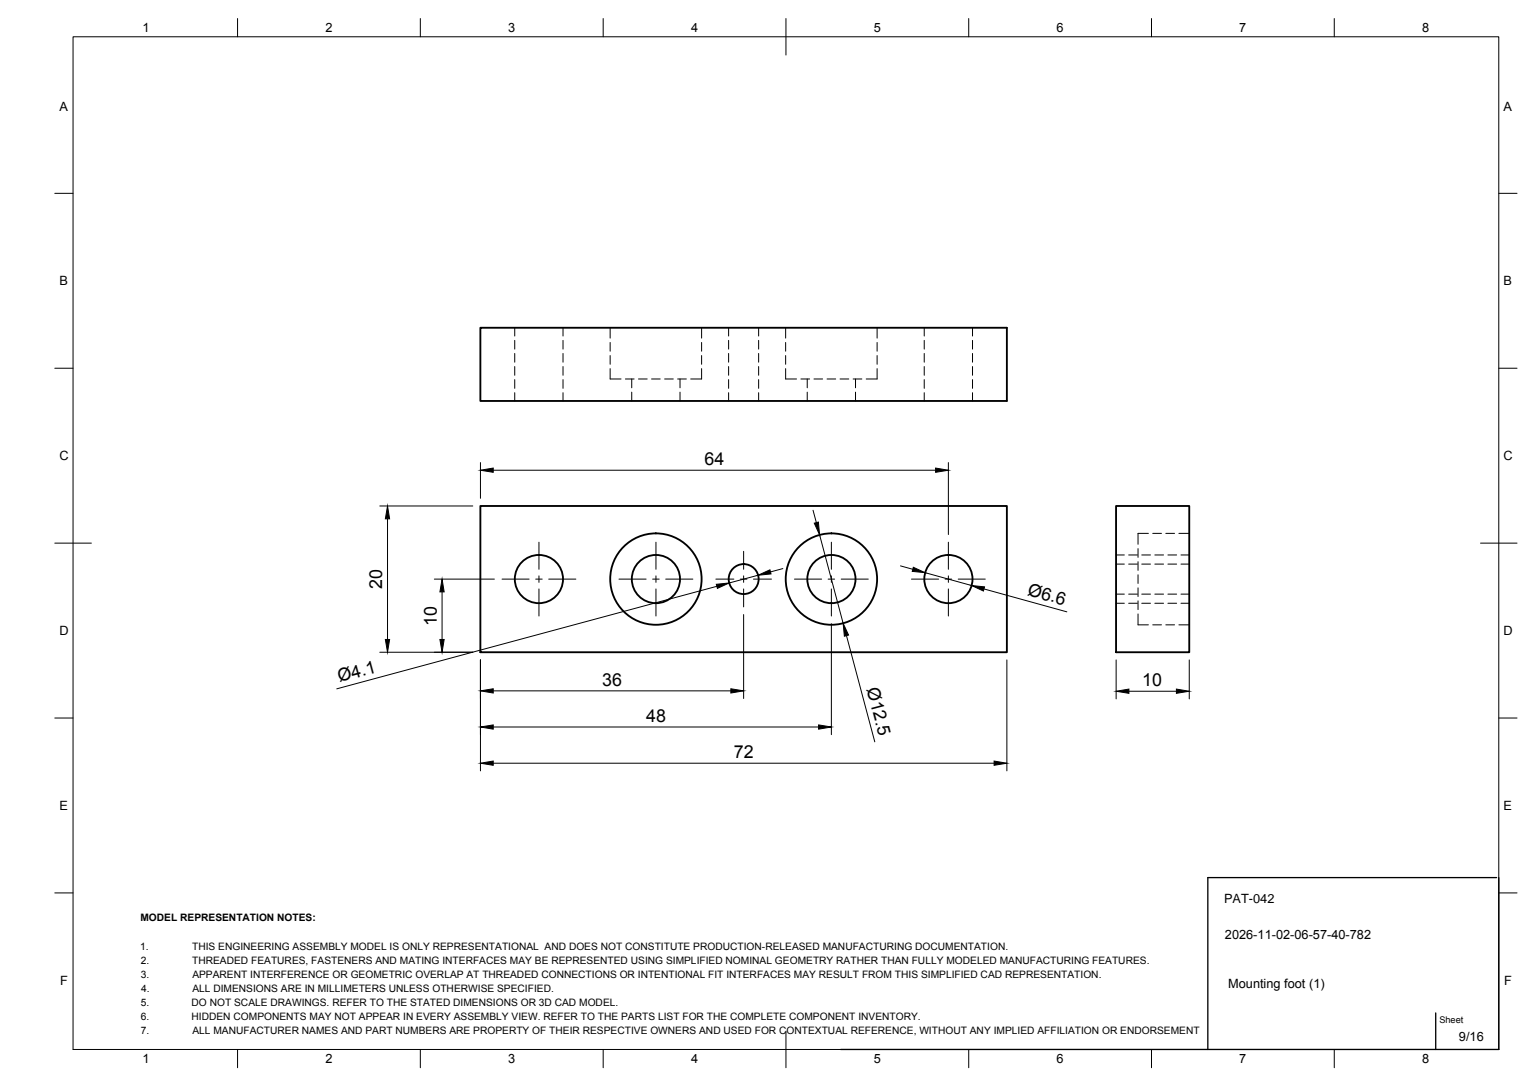
ISO-10303-21;
HEADER;
/* Generated by software containing ST-Developer
 * from STEP Tools, Inc. (www.steptools.com) 
 */

FILE_DESCRIPTION(
/* description */ ('Manifold and mounting hardware'),
/* implementation_level */ '2;1');

FILE_NAME(
/* name */ 'Mounting foot (1).step',
/* time_stamp */ '2026-10-28T21:46:49-07:00',
/* author */ (''),
/* organization */ (''),
/* preprocessor_version */ 'ST-DEVELOPER v20.2',
/* originating_system */ 'Autodesk Translation Framework v15.17.0.0',
/* authorisation */ '');

FILE_SCHEMA (('AUTOMOTIVE_DESIGN { 1 0 10303 214 3 1 1 }'));
ENDSEC;

DATA;
#10=MECHANICAL_DESIGN_GEOMETRIC_PRESENTATION_REPRESENTATION('',(#156),#5638);
#128=SHAPE_REPRESENTATION_RELATIONSHIP('SRR','None',#5707,#142);
#142=ADVANCED_BREP_SHAPE_REPRESENTATION('',(#170),#5629);
#156=STYLED_ITEM('',(#5853),#170);
#170=MANIFOLD_SOLID_BREP('Body1',#3146);
#224=FACE_BOUND('',#671,.T.);
#225=FACE_BOUND('',#674,.T.);
#226=FACE_BOUND('',#682,.T.);
#227=FACE_BOUND('',#683,.T.);
#228=FACE_BOUND('',#684,.T.);
#229=FACE_BOUND('',#685,.T.);
#230=FACE_BOUND('',#686,.T.);
#231=FACE_BOUND('',#688,.T.);
#232=FACE_BOUND('',#689,.T.);
#233=FACE_BOUND('',#690,.T.);
#234=FACE_BOUND('',#691,.T.);
#235=FACE_BOUND('',#692,.T.);
#307=CYLINDRICAL_SURFACE('',#3507,0.205);
#308=CYLINDRICAL_SURFACE('',#3510,0.33);
#309=CYLINDRICAL_SURFACE('',#3513,0.33);
#310=CYLINDRICAL_SURFACE('',#3516,0.625);
#311=CYLINDRICAL_SURFACE('',#3521,0.625);
#312=CYLINDRICAL_SURFACE('',#3526,0.33);
#313=CYLINDRICAL_SURFACE('',#3528,0.33);
#434=FACE_OUTER_BOUND('',#666,.T.);
#435=FACE_OUTER_BOUND('',#667,.T.);
#436=FACE_OUTER_BOUND('',#668,.T.);
#437=FACE_OUTER_BOUND('',#669,.T.);
#438=FACE_OUTER_BOUND('',#670,.T.);
#439=FACE_OUTER_BOUND('',#672,.T.);
#440=FACE_OUTER_BOUND('',#673,.T.);
#441=FACE_OUTER_BOUND('',#675,.T.);
#442=FACE_OUTER_BOUND('',#676,.T.);
#443=FACE_OUTER_BOUND('',#677,.T.);
#444=FACE_OUTER_BOUND('',#678,.T.);
#445=FACE_OUTER_BOUND('',#679,.T.);
#446=FACE_OUTER_BOUND('',#680,.T.);
#447=FACE_OUTER_BOUND('',#681,.T.);
#448=FACE_OUTER_BOUND('',#687,.T.);
#666=EDGE_LOOP('',(#2508,#2509,#2510,#2511));
#667=EDGE_LOOP('',(#2512,#2513,#2514,#2515));
#668=EDGE_LOOP('',(#2516,#2517,#2518,#2519));
#669=EDGE_LOOP('',(#2520,#2521,#2522,#2523));
#670=EDGE_LOOP('',(#2524));
#671=EDGE_LOOP('',(#2525));
#672=EDGE_LOOP('',(#2526,#2527,#2528,#2529));
#673=EDGE_LOOP('',(#2530));
#674=EDGE_LOOP('',(#2531));
#675=EDGE_LOOP('',(#2532,#2533,#2534,#2535));
#676=EDGE_LOOP('',(#2536,#2537,#2538,#2539));
#677=EDGE_LOOP('',(#2540,#2541,#2542,#2543));
#678=EDGE_LOOP('',(#2544,#2545,#2546,#2547));
#679=EDGE_LOOP('',(#2548,#2549,#2550,#2551));
#680=EDGE_LOOP('',(#2552,#2553,#2554,#2555));
#681=EDGE_LOOP('',(#2556,#2557,#2558,#2559));
#682=EDGE_LOOP('',(#2560));
#683=EDGE_LOOP('',(#2561));
#684=EDGE_LOOP('',(#2562));
#685=EDGE_LOOP('',(#2563));
#686=EDGE_LOOP('',(#2564));
#687=EDGE_LOOP('',(#2565,#2566,#2567,#2568));
#688=EDGE_LOOP('',(#2569));
#689=EDGE_LOOP('',(#2570));
#690=EDGE_LOOP('',(#2571));
#691=EDGE_LOOP('',(#2572));
#692=EDGE_LOOP('',(#2573));
#847=CIRCLE('',#3508,0.205);
#848=CIRCLE('',#3509,0.205);
#849=CIRCLE('',#3511,0.33);
#850=CIRCLE('',#3512,0.33);
#851=CIRCLE('',#3514,0.33);
#852=CIRCLE('',#3515,0.33);
#853=CIRCLE('',#3517,0.625);
#854=CIRCLE('',#3518,0.625);
#855=CIRCLE('',#3520,0.33);
#856=CIRCLE('',#3522,0.625);
#857=CIRCLE('',#3523,0.625);
#858=CIRCLE('',#3525,0.33);
#859=CIRCLE('',#3527,0.33);
#860=CIRCLE('',#3529,0.33);
#1039=LINE('',#5215,#1286);
#1040=LINE('',#5221,#1287);
#1041=LINE('',#5227,#1288);
#1042=LINE('',#5233,#1289);
#1043=LINE('',#5242,#1290);
#1044=LINE('',#5249,#1291);
#1045=LINE('',#5253,#1292);
#1046=LINE('',#5258,#1293);
#1047=LINE('',#5260,#1294);
#1048=LINE('',#5262,#1295);
#1049=LINE('',#5263,#1296);
#1050=LINE('',#5266,#1297);
#1051=LINE('',#5268,#1298);
#1052=LINE('',#5269,#1299);
#1053=LINE('',#5272,#1300);
#1054=LINE('',#5274,#1301);
#1055=LINE('',#5275,#1302);
#1056=LINE('',#5277,#1303);
#1057=LINE('',#5278,#1304);
#1286=VECTOR('',#4214,0.205);
#1287=VECTOR('',#4221,0.33);
#1288=VECTOR('',#4228,0.33);
#1289=VECTOR('',#4235,0.625);
#1290=VECTOR('',#4246,0.625);
#1291=VECTOR('',#4255,0.33);
#1292=VECTOR('',#4260,0.33);
#1293=VECTOR('',#4265,1.);
#1294=VECTOR('',#4266,1.);
#1295=VECTOR('',#4267,1.);
#1296=VECTOR('',#4268,1.);
#1297=VECTOR('',#4271,1.);
#1298=VECTOR('',#4272,1.);
#1299=VECTOR('',#4273,1.);
#1300=VECTOR('',#4276,1.);
#1301=VECTOR('',#4277,1.);
#1302=VECTOR('',#4278,1.);
#1303=VECTOR('',#4281,1.);
#1304=VECTOR('',#4282,1.);
#1545=VERTEX_POINT('',#5212);
#1546=VERTEX_POINT('',#5214);
#1547=VERTEX_POINT('',#5218);
#1548=VERTEX_POINT('',#5220);
#1549=VERTEX_POINT('',#5224);
#1550=VERTEX_POINT('',#5226);
#1551=VERTEX_POINT('',#5230);
#1552=VERTEX_POINT('',#5232);
#1553=VERTEX_POINT('',#5236);
#1554=VERTEX_POINT('',#5239);
#1555=VERTEX_POINT('',#5241);
#1556=VERTEX_POINT('',#5245);
#1557=VERTEX_POINT('',#5248);
#1558=VERTEX_POINT('',#5252);
#1559=VERTEX_POINT('',#5256);
#1560=VERTEX_POINT('',#5257);
#1561=VERTEX_POINT('',#5259);
#1562=VERTEX_POINT('',#5261);
#1563=VERTEX_POINT('',#5265);
#1564=VERTEX_POINT('',#5267);
#1565=VERTEX_POINT('',#5271);
#1566=VERTEX_POINT('',#5273);
#1883=EDGE_CURVE('',#1545,#1545,#847,.T.);
#1884=EDGE_CURVE('',#1545,#1546,#1039,.T.);
#1885=EDGE_CURVE('',#1546,#1546,#848,.T.);
#1886=EDGE_CURVE('',#1547,#1547,#849,.T.);
#1887=EDGE_CURVE('',#1547,#1548,#1040,.T.);
#1888=EDGE_CURVE('',#1548,#1548,#850,.T.);
#1889=EDGE_CURVE('',#1549,#1549,#851,.T.);
#1890=EDGE_CURVE('',#1549,#1550,#1041,.T.);
#1891=EDGE_CURVE('',#1550,#1550,#852,.T.);
#1892=EDGE_CURVE('',#1551,#1551,#853,.T.);
#1893=EDGE_CURVE('',#1551,#1552,#1042,.T.);
#1894=EDGE_CURVE('',#1552,#1552,#854,.T.);
#1895=EDGE_CURVE('',#1553,#1553,#855,.T.);
#1896=EDGE_CURVE('',#1554,#1554,#856,.T.);
#1897=EDGE_CURVE('',#1554,#1555,#1043,.T.);
#1898=EDGE_CURVE('',#1555,#1555,#857,.T.);
#1899=EDGE_CURVE('',#1556,#1556,#858,.T.);
#1900=EDGE_CURVE('',#1553,#1557,#1044,.T.);
#1901=EDGE_CURVE('',#1557,#1557,#859,.T.);
#1902=EDGE_CURVE('',#1556,#1558,#1045,.T.);
#1903=EDGE_CURVE('',#1558,#1558,#860,.T.);
#1904=EDGE_CURVE('',#1559,#1560,#1046,.T.);
#1905=EDGE_CURVE('',#1560,#1561,#1047,.T.);
#1906=EDGE_CURVE('',#1562,#1561,#1048,.T.);
#1907=EDGE_CURVE('',#1559,#1562,#1049,.T.);
#1908=EDGE_CURVE('',#1563,#1559,#1050,.T.);
#1909=EDGE_CURVE('',#1564,#1562,#1051,.T.);
#1910=EDGE_CURVE('',#1563,#1564,#1052,.T.);
#1911=EDGE_CURVE('',#1565,#1563,#1053,.T.);
#1912=EDGE_CURVE('',#1566,#1564,#1054,.T.);
#1913=EDGE_CURVE('',#1565,#1566,#1055,.T.);
#1914=EDGE_CURVE('',#1560,#1565,#1056,.T.);
#1915=EDGE_CURVE('',#1561,#1566,#1057,.T.);
#2508=ORIENTED_EDGE('',*,*,#1883,.F.);
#2509=ORIENTED_EDGE('',*,*,#1884,.T.);
#2510=ORIENTED_EDGE('',*,*,#1885,.F.);
#2511=ORIENTED_EDGE('',*,*,#1884,.F.);
#2512=ORIENTED_EDGE('',*,*,#1886,.F.);
#2513=ORIENTED_EDGE('',*,*,#1887,.T.);
#2514=ORIENTED_EDGE('',*,*,#1888,.F.);
#2515=ORIENTED_EDGE('',*,*,#1887,.F.);
#2516=ORIENTED_EDGE('',*,*,#1889,.F.);
#2517=ORIENTED_EDGE('',*,*,#1890,.T.);
#2518=ORIENTED_EDGE('',*,*,#1891,.F.);
#2519=ORIENTED_EDGE('',*,*,#1890,.F.);
#2520=ORIENTED_EDGE('',*,*,#1892,.F.);
#2521=ORIENTED_EDGE('',*,*,#1893,.T.);
#2522=ORIENTED_EDGE('',*,*,#1894,.T.);
#2523=ORIENTED_EDGE('',*,*,#1893,.F.);
#2524=ORIENTED_EDGE('',*,*,#1894,.F.);
#2525=ORIENTED_EDGE('',*,*,#1895,.F.);
#2526=ORIENTED_EDGE('',*,*,#1896,.F.);
#2527=ORIENTED_EDGE('',*,*,#1897,.T.);
#2528=ORIENTED_EDGE('',*,*,#1898,.T.);
#2529=ORIENTED_EDGE('',*,*,#1897,.F.);
#2530=ORIENTED_EDGE('',*,*,#1898,.F.);
#2531=ORIENTED_EDGE('',*,*,#1899,.F.);
#2532=ORIENTED_EDGE('',*,*,#1895,.T.);
#2533=ORIENTED_EDGE('',*,*,#1900,.T.);
#2534=ORIENTED_EDGE('',*,*,#1901,.F.);
#2535=ORIENTED_EDGE('',*,*,#1900,.F.);
#2536=ORIENTED_EDGE('',*,*,#1899,.T.);
#2537=ORIENTED_EDGE('',*,*,#1902,.T.);
#2538=ORIENTED_EDGE('',*,*,#1903,.F.);
#2539=ORIENTED_EDGE('',*,*,#1902,.F.);
#2540=ORIENTED_EDGE('',*,*,#1904,.T.);
#2541=ORIENTED_EDGE('',*,*,#1905,.T.);
#2542=ORIENTED_EDGE('',*,*,#1906,.F.);
#2543=ORIENTED_EDGE('',*,*,#1907,.F.);
#2544=ORIENTED_EDGE('',*,*,#1908,.T.);
#2545=ORIENTED_EDGE('',*,*,#1907,.T.);
#2546=ORIENTED_EDGE('',*,*,#1909,.F.);
#2547=ORIENTED_EDGE('',*,*,#1910,.F.);
#2548=ORIENTED_EDGE('',*,*,#1911,.T.);
#2549=ORIENTED_EDGE('',*,*,#1910,.T.);
#2550=ORIENTED_EDGE('',*,*,#1912,.F.);
#2551=ORIENTED_EDGE('',*,*,#1913,.F.);
#2552=ORIENTED_EDGE('',*,*,#1914,.T.);
#2553=ORIENTED_EDGE('',*,*,#1913,.T.);
#2554=ORIENTED_EDGE('',*,*,#1915,.F.);
#2555=ORIENTED_EDGE('',*,*,#1905,.F.);
#2556=ORIENTED_EDGE('',*,*,#1915,.T.);
#2557=ORIENTED_EDGE('',*,*,#1912,.T.);
#2558=ORIENTED_EDGE('',*,*,#1909,.T.);
#2559=ORIENTED_EDGE('',*,*,#1906,.T.);
#2560=ORIENTED_EDGE('',*,*,#1885,.T.);
#2561=ORIENTED_EDGE('',*,*,#1888,.T.);
#2562=ORIENTED_EDGE('',*,*,#1891,.T.);
#2563=ORIENTED_EDGE('',*,*,#1901,.T.);
#2564=ORIENTED_EDGE('',*,*,#1903,.T.);
#2565=ORIENTED_EDGE('',*,*,#1914,.F.);
#2566=ORIENTED_EDGE('',*,*,#1904,.F.);
#2567=ORIENTED_EDGE('',*,*,#1908,.F.);
#2568=ORIENTED_EDGE('',*,*,#1911,.F.);
#2569=ORIENTED_EDGE('',*,*,#1883,.T.);
#2570=ORIENTED_EDGE('',*,*,#1886,.T.);
#2571=ORIENTED_EDGE('',*,*,#1889,.T.);
#2572=ORIENTED_EDGE('',*,*,#1892,.T.);
#2573=ORIENTED_EDGE('',*,*,#1896,.T.);
#2900=PLANE('',#3519);
#2901=PLANE('',#3524);
#2902=PLANE('',#3530);
#2903=PLANE('',#3531);
#2904=PLANE('',#3532);
#2905=PLANE('',#3533);
#2906=PLANE('',#3534);
#2907=PLANE('',#3535);
#3058=ADVANCED_FACE('',(#434),#307,.F.);
#3059=ADVANCED_FACE('',(#435),#308,.F.);
#3060=ADVANCED_FACE('',(#436),#309,.F.);
#3061=ADVANCED_FACE('',(#437),#310,.F.);
#3062=ADVANCED_FACE('',(#438,#224),#2900,.F.);
#3063=ADVANCED_FACE('',(#439),#311,.F.);
#3064=ADVANCED_FACE('',(#440,#225),#2901,.F.);
#3065=ADVANCED_FACE('',(#441),#312,.F.);
#3066=ADVANCED_FACE('',(#442),#313,.F.);
#3067=ADVANCED_FACE('',(#443),#2902,.T.);
#3068=ADVANCED_FACE('',(#444),#2903,.T.);
#3069=ADVANCED_FACE('',(#445),#2904,.T.);
#3070=ADVANCED_FACE('',(#446),#2905,.T.);
#3071=ADVANCED_FACE('',(#447,#226,#227,#228,#229,#230),#2906,.T.);
#3072=ADVANCED_FACE('',(#448,#231,#232,#233,#234,#235),#2907,.F.);
#3146=CLOSED_SHELL('',(#3058,#3059,#3060,#3061,#3062,#3063,#3064,#3065,
#3066,#3067,#3068,#3069,#3070,#3071,#3072));
#3506=AXIS2_PLACEMENT_3D('',#5210,#4208,#4209);
#3507=AXIS2_PLACEMENT_3D('',#5211,#4210,#4211);
#3508=AXIS2_PLACEMENT_3D('',#5213,#4212,#4213);
#3509=AXIS2_PLACEMENT_3D('',#5216,#4215,#4216);
#3510=AXIS2_PLACEMENT_3D('',#5217,#4217,#4218);
#3511=AXIS2_PLACEMENT_3D('',#5219,#4219,#4220);
#3512=AXIS2_PLACEMENT_3D('',#5222,#4222,#4223);
#3513=AXIS2_PLACEMENT_3D('',#5223,#4224,#4225);
#3514=AXIS2_PLACEMENT_3D('',#5225,#4226,#4227);
#3515=AXIS2_PLACEMENT_3D('',#5228,#4229,#4230);
#3516=AXIS2_PLACEMENT_3D('',#5229,#4231,#4232);
#3517=AXIS2_PLACEMENT_3D('',#5231,#4233,#4234);
#3518=AXIS2_PLACEMENT_3D('',#5234,#4236,#4237);
#3519=AXIS2_PLACEMENT_3D('',#5235,#4238,#4239);
#3520=AXIS2_PLACEMENT_3D('',#5237,#4240,#4241);
#3521=AXIS2_PLACEMENT_3D('',#5238,#4242,#4243);
#3522=AXIS2_PLACEMENT_3D('',#5240,#4244,#4245);
#3523=AXIS2_PLACEMENT_3D('',#5243,#4247,#4248);
#3524=AXIS2_PLACEMENT_3D('',#5244,#4249,#4250);
#3525=AXIS2_PLACEMENT_3D('',#5246,#4251,#4252);
#3526=AXIS2_PLACEMENT_3D('',#5247,#4253,#4254);
#3527=AXIS2_PLACEMENT_3D('',#5250,#4256,#4257);
#3528=AXIS2_PLACEMENT_3D('',#5251,#4258,#4259);
#3529=AXIS2_PLACEMENT_3D('',#5254,#4261,#4262);
#3530=AXIS2_PLACEMENT_3D('',#5255,#4263,#4264);
#3531=AXIS2_PLACEMENT_3D('',#5264,#4269,#4270);
#3532=AXIS2_PLACEMENT_3D('',#5270,#4274,#4275);
#3533=AXIS2_PLACEMENT_3D('',#5276,#4279,#4280);
#3534=AXIS2_PLACEMENT_3D('',#5279,#4283,#4284);
#3535=AXIS2_PLACEMENT_3D('',#5280,#4285,#4286);
#4208=DIRECTION('axis',(0.,0.,1.));
#4209=DIRECTION('refdir',(1.,0.,0.));
#4210=DIRECTION('center_axis',(0.,0.,1.));
#4211=DIRECTION('ref_axis',(1.,0.,0.));
#4212=DIRECTION('center_axis',(0.,0.,1.));
#4213=DIRECTION('ref_axis',(1.,0.,0.));
#4214=DIRECTION('',(0.,0.,1.));
#4215=DIRECTION('center_axis',(0.,0.,-1.));
#4216=DIRECTION('ref_axis',(1.,0.,0.));
#4217=DIRECTION('center_axis',(0.,0.,1.));
#4218=DIRECTION('ref_axis',(1.,0.,0.));
#4219=DIRECTION('center_axis',(0.,0.,1.));
#4220=DIRECTION('ref_axis',(1.,0.,0.));
#4221=DIRECTION('',(0.,0.,1.));
#4222=DIRECTION('center_axis',(0.,0.,-1.));
#4223=DIRECTION('ref_axis',(1.,0.,0.));
#4224=DIRECTION('center_axis',(0.,0.,1.));
#4225=DIRECTION('ref_axis',(1.,0.,0.));
#4226=DIRECTION('center_axis',(0.,0.,1.));
#4227=DIRECTION('ref_axis',(1.,0.,0.));
#4228=DIRECTION('',(0.,0.,1.));
#4229=DIRECTION('center_axis',(0.,0.,-1.));
#4230=DIRECTION('ref_axis',(1.,0.,0.));
#4231=DIRECTION('center_axis',(0.,0.,1.));
#4232=DIRECTION('ref_axis',(1.,0.,0.));
#4233=DIRECTION('center_axis',(0.,0.,1.));
#4234=DIRECTION('ref_axis',(1.,0.,0.));
#4235=DIRECTION('',(0.,0.,1.));
#4236=DIRECTION('center_axis',(0.,0.,1.));
#4237=DIRECTION('ref_axis',(1.,0.,0.));
#4238=DIRECTION('center_axis',(0.,0.,1.));
#4239=DIRECTION('ref_axis',(1.,0.,0.));
#4240=DIRECTION('center_axis',(0.,0.,-1.));
#4241=DIRECTION('ref_axis',(1.,0.,0.));
#4242=DIRECTION('center_axis',(0.,0.,1.));
#4243=DIRECTION('ref_axis',(1.,0.,0.));
#4244=DIRECTION('center_axis',(0.,0.,1.));
#4245=DIRECTION('ref_axis',(1.,0.,0.));
#4246=DIRECTION('',(0.,0.,1.));
#4247=DIRECTION('center_axis',(0.,0.,1.));
#4248=DIRECTION('ref_axis',(1.,0.,0.));
#4249=DIRECTION('center_axis',(0.,0.,1.));
#4250=DIRECTION('ref_axis',(1.,0.,0.));
#4251=DIRECTION('center_axis',(0.,0.,-1.));
#4252=DIRECTION('ref_axis',(1.,0.,0.));
#4253=DIRECTION('center_axis',(0.,0.,1.));
#4254=DIRECTION('ref_axis',(1.,0.,0.));
#4255=DIRECTION('',(0.,0.,1.));
#4256=DIRECTION('center_axis',(0.,0.,-1.));
#4257=DIRECTION('ref_axis',(1.,0.,0.));
#4258=DIRECTION('center_axis',(0.,0.,1.));
#4259=DIRECTION('ref_axis',(1.,0.,0.));
#4260=DIRECTION('',(0.,0.,1.));
#4261=DIRECTION('center_axis',(0.,0.,-1.));
#4262=DIRECTION('ref_axis',(1.,0.,0.));
#4263=DIRECTION('center_axis',(0.,1.,0.));
#4264=DIRECTION('ref_axis',(-1.,0.,0.));
#4265=DIRECTION('',(-1.,0.,0.));
#4266=DIRECTION('',(0.,0.,1.));
#4267=DIRECTION('',(-1.,0.,0.));
#4268=DIRECTION('',(0.,0.,1.));
#4269=DIRECTION('center_axis',(1.,0.,0.));
#4270=DIRECTION('ref_axis',(0.,1.,0.));
#4271=DIRECTION('',(0.,1.,0.));
#4272=DIRECTION('',(0.,1.,0.));
#4273=DIRECTION('',(0.,0.,1.));
#4274=DIRECTION('center_axis',(0.,-1.,0.));
#4275=DIRECTION('ref_axis',(1.,0.,0.));
#4276=DIRECTION('',(1.,0.,0.));
#4277=DIRECTION('',(1.,0.,0.));
#4278=DIRECTION('',(0.,0.,1.));
#4279=DIRECTION('center_axis',(-1.,0.,0.));
#4280=DIRECTION('ref_axis',(0.,-1.,0.));
#4281=DIRECTION('',(0.,-1.,0.));
#4282=DIRECTION('',(0.,-1.,0.));
#4283=DIRECTION('center_axis',(0.,0.,1.));
#4284=DIRECTION('ref_axis',(1.,0.,0.));
#4285=DIRECTION('center_axis',(0.,0.,1.));
#4286=DIRECTION('ref_axis',(1.,0.,0.));
#5210=CARTESIAN_POINT('',(0.,0.,0.));
#5211=CARTESIAN_POINT('Origin',(4.5,0.,0.9));
#5212=CARTESIAN_POINT('',(4.295,-2.51052593825207E-17,1.));
#5213=CARTESIAN_POINT('Origin',(4.5,0.,1.));
#5214=CARTESIAN_POINT('',(4.295,2.51052593825207E-17,2.));
#5215=CARTESIAN_POINT('',(4.295,-2.51052593825207E-17,0.9));
#5216=CARTESIAN_POINT('Origin',(4.5,0.,2.));
#5217=CARTESIAN_POINT('Origin',(4.5,-2.8,0.9));
#5218=CARTESIAN_POINT('',(4.17,-2.8,1.));
#5219=CARTESIAN_POINT('Origin',(4.5,-2.8,1.));
#5220=CARTESIAN_POINT('',(4.17,-2.8,2.));
#5221=CARTESIAN_POINT('',(4.17,-2.8,0.9));
#5222=CARTESIAN_POINT('Origin',(4.5,-2.8,2.));
#5223=CARTESIAN_POINT('Origin',(4.5,2.8,0.9));
#5224=CARTESIAN_POINT('',(4.17,2.8,1.));
#5225=CARTESIAN_POINT('Origin',(4.5,2.8,1.));
#5226=CARTESIAN_POINT('',(4.17,2.8,2.));
#5227=CARTESIAN_POINT('',(4.17,2.8,0.9));
#5228=CARTESIAN_POINT('Origin',(4.5,2.8,2.));
#5229=CARTESIAN_POINT('Origin',(4.5,-1.2,0.9));
#5230=CARTESIAN_POINT('',(3.875,-1.2,1.));
#5231=CARTESIAN_POINT('Origin',(4.5,-1.2,1.));
#5232=CARTESIAN_POINT('',(3.875,-1.2,1.7));
#5233=CARTESIAN_POINT('',(3.875,-1.2,0.9));
#5234=CARTESIAN_POINT('Origin',(4.5,-1.2,1.7));
#5235=CARTESIAN_POINT('Origin',(4.5,-1.2,1.7));
#5236=CARTESIAN_POINT('',(4.17,-1.2,1.7));
#5237=CARTESIAN_POINT('Origin',(4.5,-1.2,1.7));
#5238=CARTESIAN_POINT('Origin',(4.5,1.2,0.9));
#5239=CARTESIAN_POINT('',(3.875,1.2,1.));
#5240=CARTESIAN_POINT('Origin',(4.5,1.2,1.));
#5241=CARTESIAN_POINT('',(3.875,1.2,1.7));
#5242=CARTESIAN_POINT('',(3.875,1.2,0.9));
#5243=CARTESIAN_POINT('Origin',(4.5,1.2,1.7));
#5244=CARTESIAN_POINT('Origin',(4.5,1.2,1.7));
#5245=CARTESIAN_POINT('',(4.17,1.2,1.7));
#5246=CARTESIAN_POINT('Origin',(4.5,1.2,1.7));
#5247=CARTESIAN_POINT('Origin',(4.5,-1.2,0.9));
#5248=CARTESIAN_POINT('',(4.17,-1.2,2.));
#5249=CARTESIAN_POINT('',(4.17,-1.2,0.9));
#5250=CARTESIAN_POINT('Origin',(4.5,-1.2,2.));
#5251=CARTESIAN_POINT('Origin',(4.5,1.2,0.9));
#5252=CARTESIAN_POINT('',(4.17,1.2,2.));
#5253=CARTESIAN_POINT('',(4.17,1.2,0.9));
#5254=CARTESIAN_POINT('Origin',(4.5,1.2,2.));
#5255=CARTESIAN_POINT('Origin',(5.5,3.6,1.));
#5256=CARTESIAN_POINT('',(5.5,3.6,1.));
#5257=CARTESIAN_POINT('',(3.5,3.6,1.));
#5258=CARTESIAN_POINT('',(5.5,3.6,1.));
#5259=CARTESIAN_POINT('',(3.5,3.6,2.));
#5260=CARTESIAN_POINT('',(3.5,3.6,1.));
#5261=CARTESIAN_POINT('',(5.5,3.6,2.));
#5262=CARTESIAN_POINT('',(5.5,3.6,2.));
#5263=CARTESIAN_POINT('',(5.5,3.6,1.));
#5264=CARTESIAN_POINT('Origin',(5.5,-3.6,1.));
#5265=CARTESIAN_POINT('',(5.5,-3.6,1.));
#5266=CARTESIAN_POINT('',(5.5,-3.6,1.));
#5267=CARTESIAN_POINT('',(5.5,-3.6,2.));
#5268=CARTESIAN_POINT('',(5.5,-3.6,2.));
#5269=CARTESIAN_POINT('',(5.5,-3.6,1.));
#5270=CARTESIAN_POINT('Origin',(3.5,-3.6,1.));
#5271=CARTESIAN_POINT('',(3.5,-3.6,1.));
#5272=CARTESIAN_POINT('',(3.5,-3.6,1.));
#5273=CARTESIAN_POINT('',(3.5,-3.6,2.));
#5274=CARTESIAN_POINT('',(3.5,-3.6,2.));
#5275=CARTESIAN_POINT('',(3.5,-3.6,1.));
#5276=CARTESIAN_POINT('Origin',(3.5,3.6,1.));
#5277=CARTESIAN_POINT('',(3.5,3.6,1.));
#5278=CARTESIAN_POINT('',(3.5,3.6,2.));
#5279=CARTESIAN_POINT('Origin',(4.5,0.,2.));
#5280=CARTESIAN_POINT('Origin',(4.5,0.,1.));
#5612=UNCERTAINTY_MEASURE_WITH_UNIT(LENGTH_MEASURE(0.001),#5639,
'DISTANCE_ACCURACY_VALUE',
'Maximum model space distance between geometric entities at asserted c
onnectivities');
#5621=UNCERTAINTY_MEASURE_WITH_UNIT(LENGTH_MEASURE(0.001),#5639,
'DISTANCE_ACCURACY_VALUE',
'Maximum model space distance between geometric entities at asserted c
onnectivities');
#5629=(
GEOMETRIC_REPRESENTATION_CONTEXT(3)
GLOBAL_UNCERTAINTY_ASSIGNED_CONTEXT((#5612))
GLOBAL_UNIT_ASSIGNED_CONTEXT((#5639,#5641,#5642))
REPRESENTATION_CONTEXT('','3D')
);
#5638=(
GEOMETRIC_REPRESENTATION_CONTEXT(3)
GLOBAL_UNCERTAINTY_ASSIGNED_CONTEXT((#5621))
GLOBAL_UNIT_ASSIGNED_CONTEXT((#5639,#5641,#5642))
REPRESENTATION_CONTEXT('','3D')
);
#5639=(
LENGTH_UNIT()
NAMED_UNIT(*)
SI_UNIT(.CENTI.,.METRE.)
);
#5641=(
NAMED_UNIT(*)
PLANE_ANGLE_UNIT()
SI_UNIT($,.RADIAN.)
);
#5642=(
NAMED_UNIT(*)
SI_UNIT($,.STERADIAN.)
SOLID_ANGLE_UNIT()
);
#5650=SHAPE_DEFINITION_REPRESENTATION(#5666,#5707);
#5666=PRODUCT_DEFINITION_SHAPE('',$,#5724);
#5707=SHAPE_REPRESENTATION('',(#3506),#5629);
#5716=PRODUCT_DEFINITION_CONTEXT('part definition',#5766,'design');
#5724=PRODUCT_DEFINITION('Mounting foot (1)','Mounting foot (1)',
#5740,#5716);
#5740=PRODUCT_DEFINITION_FORMATION('',$,#5775);
#5766=APPLICATION_CONTEXT(
'Core Data for Automotive Mechanical Design Process');
#5767=PRODUCT_CONTEXT('part definition',#5766,'mechanical');
#5775=PRODUCT('Mounting foot (1)','Mounting foot (1)',
'Mounting foot (1)',(#5767));
#5847=COLOUR_RGB('Sky Blue',0.24,0.69,0.87);
#5848=FILL_AREA_STYLE_COLOUR('',#5847);
#5849=FILL_AREA_STYLE('',(#5848));
#5850=SURFACE_STYLE_FILL_AREA(#5849);
#5851=SURFACE_SIDE_STYLE('',(#5850));
#5852=SURFACE_STYLE_USAGE(.BOTH.,#5851);
#5853=PRESENTATION_STYLE_ASSIGNMENT((#5852));
ENDSEC;
END-ISO-10303-21;
